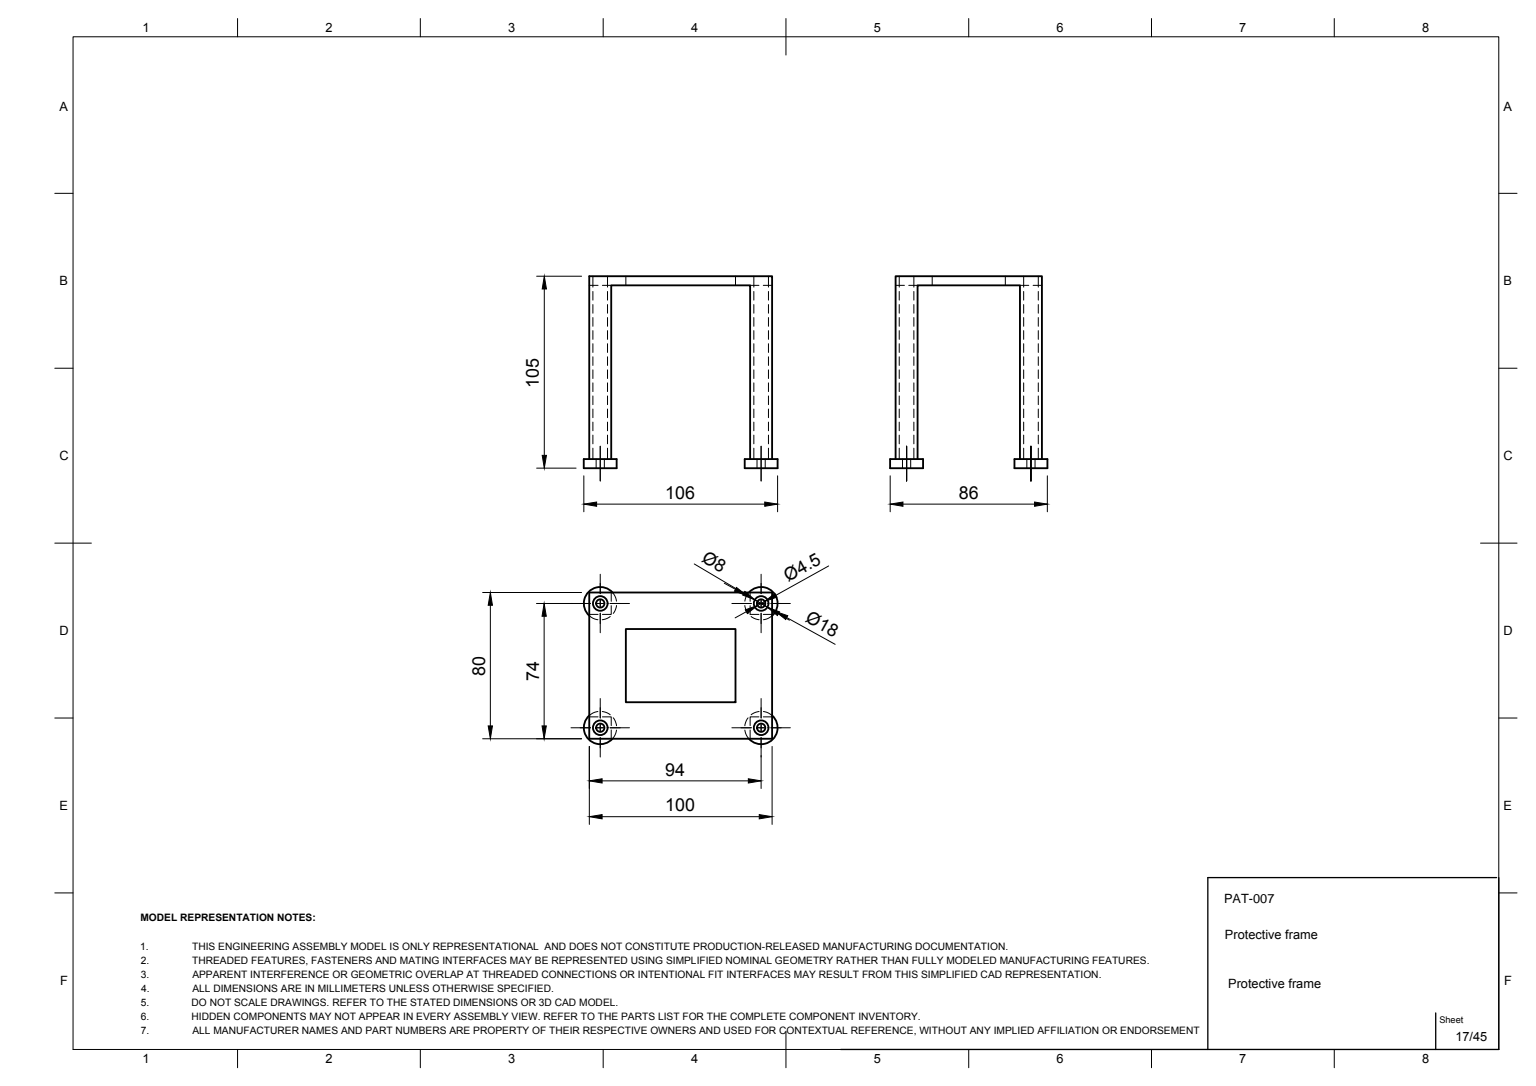
ISO-10303-21;
HEADER;
/* Generated by software containing ST-Developer
 * from STEP Tools, Inc. (www.steptools.com) 
 */

FILE_DESCRIPTION(
/* description */ ('Bearing friction torque test rig'),
/* implementation_level */ '2;1');

FILE_NAME(
/* name */ 'Protective frame.step',
/* time_stamp */ '2026-10-28T03:24:04-07:00',
/* author */ (''),
/* organization */ (''),
/* preprocessor_version */ 'ST-DEVELOPER v20.2',
/* originating_system */ 'Autodesk Translation Framework v15.17.0.0',
/* authorisation */ '');

FILE_SCHEMA (('AUTOMOTIVE_DESIGN { 1 0 10303 214 3 1 1 }'));
ENDSEC;

DATA;
#10=MECHANICAL_DESIGN_GEOMETRIC_PRESENTATION_REPRESENTATION('',(#551),#14822);
#473=SHAPE_REPRESENTATION_RELATIONSHIP('SRR','None',#15012,#512);
#512=ADVANCED_BREP_SHAPE_REPRESENTATION('',(#605),#14792);
#551=STYLED_ITEM('',(#15263),#605);
#605=MANIFOLD_SOLID_BREP('Body1',#7667);
#795=FACE_BOUND('',#1864,.T.);
#796=FACE_BOUND('',#1867,.T.);
#797=FACE_BOUND('',#1873,.T.);
#798=FACE_BOUND('',#1876,.T.);
#799=FACE_BOUND('',#1882,.T.);
#800=FACE_BOUND('',#1885,.T.);
#801=FACE_BOUND('',#1891,.T.);
#802=FACE_BOUND('',#1894,.T.);
#803=FACE_BOUND('',#1904,.T.);
#804=FACE_BOUND('',#1907,.T.);
#805=FACE_BOUND('',#1909,.T.);
#806=FACE_BOUND('',#1911,.T.);
#807=FACE_BOUND('',#1914,.T.);
#808=FACE_BOUND('',#1917,.T.);
#809=FACE_BOUND('',#1918,.T.);
#810=FACE_BOUND('',#1919,.T.);
#811=FACE_BOUND('',#1920,.T.);
#812=FACE_BOUND('',#1921,.T.);
#949=PLANE('',#8521);
#950=PLANE('',#8525);
#951=PLANE('',#8529);
#952=PLANE('',#8530);
#953=PLANE('',#8534);
#954=PLANE('',#8538);
#955=PLANE('',#8542);
#956=PLANE('',#8543);
#957=PLANE('',#8547);
#958=PLANE('',#8551);
#959=PLANE('',#8555);
#960=PLANE('',#8556);
#961=PLANE('',#8560);
#962=PLANE('',#8564);
#963=PLANE('',#8568);
#964=PLANE('',#8569);
#965=PLANE('',#8570);
#966=PLANE('',#8571);
#967=PLANE('',#8572);
#968=PLANE('',#8573);
#969=PLANE('',#8574);
#970=PLANE('',#8575);
#971=PLANE('',#8576);
#972=PLANE('',#8577);
#973=PLANE('',#8578);
#974=PLANE('',#8579);
#975=PLANE('',#8580);
#976=PLANE('',#8581);
#977=PLANE('',#8582);
#978=PLANE('',#8583);
#1266=FACE_OUTER_BOUND('',#1862,.T.);
#1267=FACE_OUTER_BOUND('',#1863,.T.);
#1268=FACE_OUTER_BOUND('',#1865,.T.);
#1269=FACE_OUTER_BOUND('',#1866,.T.);
#1270=FACE_OUTER_BOUND('',#1868,.T.);
#1271=FACE_OUTER_BOUND('',#1869,.T.);
#1272=FACE_OUTER_BOUND('',#1870,.T.);
#1273=FACE_OUTER_BOUND('',#1871,.T.);
#1274=FACE_OUTER_BOUND('',#1872,.T.);
#1275=FACE_OUTER_BOUND('',#1874,.T.);
#1276=FACE_OUTER_BOUND('',#1875,.T.);
#1277=FACE_OUTER_BOUND('',#1877,.T.);
#1278=FACE_OUTER_BOUND('',#1878,.T.);
#1279=FACE_OUTER_BOUND('',#1879,.T.);
#1280=FACE_OUTER_BOUND('',#1880,.T.);
#1281=FACE_OUTER_BOUND('',#1881,.T.);
#1282=FACE_OUTER_BOUND('',#1883,.T.);
#1283=FACE_OUTER_BOUND('',#1884,.T.);
#1284=FACE_OUTER_BOUND('',#1886,.T.);
#1285=FACE_OUTER_BOUND('',#1887,.T.);
#1286=FACE_OUTER_BOUND('',#1888,.T.);
#1287=FACE_OUTER_BOUND('',#1889,.T.);
#1288=FACE_OUTER_BOUND('',#1890,.T.);
#1289=FACE_OUTER_BOUND('',#1892,.T.);
#1290=FACE_OUTER_BOUND('',#1893,.T.);
#1291=FACE_OUTER_BOUND('',#1895,.T.);
#1292=FACE_OUTER_BOUND('',#1896,.T.);
#1293=FACE_OUTER_BOUND('',#1897,.T.);
#1294=FACE_OUTER_BOUND('',#1898,.T.);
#1295=FACE_OUTER_BOUND('',#1899,.T.);
#1296=FACE_OUTER_BOUND('',#1900,.T.);
#1297=FACE_OUTER_BOUND('',#1901,.T.);
#1298=FACE_OUTER_BOUND('',#1902,.T.);
#1299=FACE_OUTER_BOUND('',#1903,.T.);
#1300=FACE_OUTER_BOUND('',#1905,.T.);
#1301=FACE_OUTER_BOUND('',#1906,.T.);
#1302=FACE_OUTER_BOUND('',#1908,.T.);
#1303=FACE_OUTER_BOUND('',#1910,.T.);
#1304=FACE_OUTER_BOUND('',#1912,.T.);
#1305=FACE_OUTER_BOUND('',#1913,.T.);
#1306=FACE_OUTER_BOUND('',#1915,.T.);
#1307=FACE_OUTER_BOUND('',#1916,.T.);
#1862=EDGE_LOOP('',(#5904,#5905,#5906,#5907));
#1863=EDGE_LOOP('',(#5908));
#1864=EDGE_LOOP('',(#5909));
#1865=EDGE_LOOP('',(#5910,#5911,#5912,#5913));
#1866=EDGE_LOOP('',(#5914));
#1867=EDGE_LOOP('',(#5915,#5916,#5917,#5918));
#1868=EDGE_LOOP('',(#5919,#5920,#5921,#5922));
#1869=EDGE_LOOP('',(#5923,#5924,#5925,#5926,#5927,#5928,#5929,#5930));
#1870=EDGE_LOOP('',(#5931,#5932,#5933,#5934,#5935,#5936,#5937,#5938));
#1871=EDGE_LOOP('',(#5939,#5940,#5941,#5942));
#1872=EDGE_LOOP('',(#5943));
#1873=EDGE_LOOP('',(#5944));
#1874=EDGE_LOOP('',(#5945,#5946,#5947,#5948));
#1875=EDGE_LOOP('',(#5949));
#1876=EDGE_LOOP('',(#5950,#5951,#5952,#5953));
#1877=EDGE_LOOP('',(#5954,#5955,#5956,#5957));
#1878=EDGE_LOOP('',(#5958,#5959,#5960,#5961));
#1879=EDGE_LOOP('',(#5962,#5963,#5964,#5965));
#1880=EDGE_LOOP('',(#5966,#5967,#5968,#5969));
#1881=EDGE_LOOP('',(#5970));
#1882=EDGE_LOOP('',(#5971));
#1883=EDGE_LOOP('',(#5972,#5973,#5974,#5975));
#1884=EDGE_LOOP('',(#5976));
#1885=EDGE_LOOP('',(#5977,#5978,#5979,#5980));
#1886=EDGE_LOOP('',(#5981,#5982,#5983,#5984));
#1887=EDGE_LOOP('',(#5985,#5986,#5987,#5988));
#1888=EDGE_LOOP('',(#5989,#5990,#5991,#5992));
#1889=EDGE_LOOP('',(#5993,#5994,#5995,#5996));
#1890=EDGE_LOOP('',(#5997));
#1891=EDGE_LOOP('',(#5998));
#1892=EDGE_LOOP('',(#5999,#6000,#6001,#6002));
#1893=EDGE_LOOP('',(#6003));
#1894=EDGE_LOOP('',(#6004,#6005,#6006,#6007));
#1895=EDGE_LOOP('',(#6008,#6009,#6010,#6011));
#1896=EDGE_LOOP('',(#6012,#6013,#6014,#6015,#6016,#6017,#6018,#6019));
#1897=EDGE_LOOP('',(#6020,#6021,#6022,#6023));
#1898=EDGE_LOOP('',(#6024,#6025,#6026,#6027));
#1899=EDGE_LOOP('',(#6028,#6029,#6030,#6031));
#1900=EDGE_LOOP('',(#6032,#6033,#6034,#6035));
#1901=EDGE_LOOP('',(#6036,#6037,#6038,#6039));
#1902=EDGE_LOOP('',(#6040,#6041,#6042,#6043));
#1903=EDGE_LOOP('',(#6044));
#1904=EDGE_LOOP('',(#6045));
#1905=EDGE_LOOP('',(#6046,#6047,#6048,#6049));
#1906=EDGE_LOOP('',(#6050,#6051,#6052,#6053,#6054,#6055,#6056,#6057,#6058,
#6059,#6060,#6061));
#1907=EDGE_LOOP('',(#6062,#6063,#6064,#6065));
#1908=EDGE_LOOP('',(#6066));
#1909=EDGE_LOOP('',(#6067));
#1910=EDGE_LOOP('',(#6068));
#1911=EDGE_LOOP('',(#6069));
#1912=EDGE_LOOP('',(#6070,#6071,#6072,#6073));
#1913=EDGE_LOOP('',(#6074));
#1914=EDGE_LOOP('',(#6075));
#1915=EDGE_LOOP('',(#6076,#6077,#6078,#6079,#6080,#6081,#6082,#6083));
#1916=EDGE_LOOP('',(#6084,#6085,#6086,#6087));
#1917=EDGE_LOOP('',(#6088));
#1918=EDGE_LOOP('',(#6089));
#1919=EDGE_LOOP('',(#6090));
#1920=EDGE_LOOP('',(#6091));
#1921=EDGE_LOOP('',(#6092,#6093,#6094,#6095));
#2403=LINE('',#12474,#2847);
#2404=LINE('',#12482,#2848);
#2405=LINE('',#12488,#2849);
#2406=LINE('',#12490,#2850);
#2407=LINE('',#12492,#2851);
#2408=LINE('',#12493,#2852);
#2409=LINE('',#12496,#2853);
#2410=LINE('',#12500,#2854);
#2411=LINE('',#12502,#2855);
#2412=LINE('',#12504,#2856);
#2413=LINE('',#12506,#2857);
#2414=LINE('',#12508,#2858);
#2415=LINE('',#12510,#2859);
#2416=LINE('',#12511,#2860);
#2417=LINE('',#12514,#2861);
#2418=LINE('',#12516,#2862);
#2419=LINE('',#12518,#2863);
#2420=LINE('',#12520,#2864);
#2421=LINE('',#12522,#2865);
#2422=LINE('',#12523,#2866);
#2423=LINE('',#12528,#2867);
#2424=LINE('',#12536,#2868);
#2425=LINE('',#12541,#2869);
#2426=LINE('',#12543,#2870);
#2427=LINE('',#12544,#2871);
#2428=LINE('',#12547,#2872);
#2429=LINE('',#12551,#2873);
#2430=LINE('',#12552,#2874);
#2431=LINE('',#12555,#2875);
#2432=LINE('',#12556,#2876);
#2433=LINE('',#12561,#2877);
#2434=LINE('',#12569,#2878);
#2435=LINE('',#12574,#2879);
#2436=LINE('',#12576,#2880);
#2437=LINE('',#12577,#2881);
#2438=LINE('',#12580,#2882);
#2439=LINE('',#12584,#2883);
#2440=LINE('',#12586,#2884);
#2441=LINE('',#12587,#2885);
#2442=LINE('',#12589,#2886);
#2443=LINE('',#12594,#2887);
#2444=LINE('',#12602,#2888);
#2445=LINE('',#12608,#2889);
#2446=LINE('',#12610,#2890);
#2447=LINE('',#12612,#2891);
#2448=LINE('',#12613,#2892);
#2449=LINE('',#12616,#2893);
#2450=LINE('',#12620,#2894);
#2451=LINE('',#12621,#2895);
#2452=LINE('',#12623,#2896);
#2453=LINE('',#12624,#2897);
#2454=LINE('',#12627,#2898);
#2455=LINE('',#12628,#2899);
#2456=LINE('',#12632,#2900);
#2457=LINE('',#12634,#2901);
#2458=LINE('',#12636,#2902);
#2459=LINE('',#12637,#2903);
#2460=LINE('',#12640,#2904);
#2461=LINE('',#12642,#2905);
#2462=LINE('',#12643,#2906);
#2463=LINE('',#12646,#2907);
#2464=LINE('',#12648,#2908);
#2465=LINE('',#12649,#2909);
#2466=LINE('',#12651,#2910);
#2467=LINE('',#12652,#2911);
#2468=LINE('',#12655,#2912);
#2469=LINE('',#12656,#2913);
#2470=LINE('',#12659,#2914);
#2471=LINE('',#12662,#2915);
#2472=LINE('',#12663,#2916);
#2473=LINE('',#12667,#2917);
#2474=LINE('',#12670,#2918);
#2847=VECTOR('',#10106,0.4);
#2848=VECTOR('',#10117,0.225);
#2849=VECTOR('',#10122,1.);
#2850=VECTOR('',#10123,1.);
#2851=VECTOR('',#10124,1.);
#2852=VECTOR('',#10125,1.);
#2853=VECTOR('',#10128,0.9);
#2854=VECTOR('',#10133,1.);
#2855=VECTOR('',#10134,1.);
#2856=VECTOR('',#10135,1.);
#2857=VECTOR('',#10136,1.);
#2858=VECTOR('',#10137,1.);
#2859=VECTOR('',#10138,1.);
#2860=VECTOR('',#10139,1.);
#2861=VECTOR('',#10142,1.);
#2862=VECTOR('',#10143,1.);
#2863=VECTOR('',#10144,1.);
#2864=VECTOR('',#10145,1.);
#2865=VECTOR('',#10146,1.);
#2866=VECTOR('',#10147,1.);
#2867=VECTOR('',#10152,0.4);
#2868=VECTOR('',#10163,0.225);
#2869=VECTOR('',#10168,1.);
#2870=VECTOR('',#10169,1.);
#2871=VECTOR('',#10170,1.);
#2872=VECTOR('',#10173,0.9);
#2873=VECTOR('',#10178,1.);
#2874=VECTOR('',#10179,1.);
#2875=VECTOR('',#10182,1.);
#2876=VECTOR('',#10183,1.);
#2877=VECTOR('',#10188,0.4);
#2878=VECTOR('',#10199,0.225);
#2879=VECTOR('',#10204,1.);
#2880=VECTOR('',#10205,1.);
#2881=VECTOR('',#10206,1.);
#2882=VECTOR('',#10209,0.9);
#2883=VECTOR('',#10214,1.);
#2884=VECTOR('',#10215,1.);
#2885=VECTOR('',#10216,1.);
#2886=VECTOR('',#10219,1.);
#2887=VECTOR('',#10224,0.4);
#2888=VECTOR('',#10235,0.225);
#2889=VECTOR('',#10240,1.);
#2890=VECTOR('',#10241,1.);
#2891=VECTOR('',#10242,1.);
#2892=VECTOR('',#10243,1.);
#2893=VECTOR('',#10246,0.9);
#2894=VECTOR('',#10251,1.);
#2895=VECTOR('',#10252,1.);
#2896=VECTOR('',#10253,1.);
#2897=VECTOR('',#10254,1.);
#2898=VECTOR('',#10257,1.);
#2899=VECTOR('',#10258,1.);
#2900=VECTOR('',#10261,1.);
#2901=VECTOR('',#10262,1.);
#2902=VECTOR('',#10263,1.);
#2903=VECTOR('',#10264,1.);
#2904=VECTOR('',#10267,1.);
#2905=VECTOR('',#10268,1.);
#2906=VECTOR('',#10269,1.);
#2907=VECTOR('',#10272,1.);
#2908=VECTOR('',#10273,1.);
#2909=VECTOR('',#10274,1.);
#2910=VECTOR('',#10277,1.);
#2911=VECTOR('',#10278,1.);
#2912=VECTOR('',#10281,1.);
#2913=VECTOR('',#10282,1.);
#2914=VECTOR('',#10287,1.);
#2915=VECTOR('',#10290,1.);
#2916=VECTOR('',#10291,1.);
#2917=VECTOR('',#10298,1.);
#2918=VECTOR('',#10303,1.);
#3295=CIRCLE('',#8519,0.4);
#3296=CIRCLE('',#8520,0.4);
#3297=CIRCLE('',#8522,0.225);
#3298=CIRCLE('',#8524,0.225);
#3299=CIRCLE('',#8526,0.9);
#3300=CIRCLE('',#8528,0.9);
#3301=CIRCLE('',#8532,0.4);
#3302=CIRCLE('',#8533,0.4);
#3303=CIRCLE('',#8535,0.225);
#3304=CIRCLE('',#8537,0.225);
#3305=CIRCLE('',#8539,0.9);
#3306=CIRCLE('',#8541,0.9);
#3307=CIRCLE('',#8545,0.4);
#3308=CIRCLE('',#8546,0.4);
#3309=CIRCLE('',#8548,0.225);
#3310=CIRCLE('',#8550,0.225);
#3311=CIRCLE('',#8552,0.9);
#3312=CIRCLE('',#8554,0.9);
#3313=CIRCLE('',#8558,0.4);
#3314=CIRCLE('',#8559,0.4);
#3315=CIRCLE('',#8561,0.225);
#3316=CIRCLE('',#8563,0.225);
#3317=CIRCLE('',#8565,0.9);
#3318=CIRCLE('',#8567,0.9);
#3805=VERTEX_POINT('',#12471);
#3806=VERTEX_POINT('',#12473);
#3807=VERTEX_POINT('',#12477);
#3808=VERTEX_POINT('',#12480);
#3809=VERTEX_POINT('',#12484);
#3810=VERTEX_POINT('',#12486);
#3811=VERTEX_POINT('',#12487);
#3812=VERTEX_POINT('',#12489);
#3813=VERTEX_POINT('',#12491);
#3814=VERTEX_POINT('',#12495);
#3815=VERTEX_POINT('',#12499);
#3816=VERTEX_POINT('',#12501);
#3817=VERTEX_POINT('',#12503);
#3818=VERTEX_POINT('',#12505);
#3819=VERTEX_POINT('',#12507);
#3820=VERTEX_POINT('',#12509);
#3821=VERTEX_POINT('',#12513);
#3822=VERTEX_POINT('',#12515);
#3823=VERTEX_POINT('',#12517);
#3824=VERTEX_POINT('',#12519);
#3825=VERTEX_POINT('',#12521);
#3826=VERTEX_POINT('',#12525);
#3827=VERTEX_POINT('',#12527);
#3828=VERTEX_POINT('',#12531);
#3829=VERTEX_POINT('',#12534);
#3830=VERTEX_POINT('',#12538);
#3831=VERTEX_POINT('',#12540);
#3832=VERTEX_POINT('',#12542);
#3833=VERTEX_POINT('',#12546);
#3834=VERTEX_POINT('',#12550);
#3835=VERTEX_POINT('',#12554);
#3836=VERTEX_POINT('',#12558);
#3837=VERTEX_POINT('',#12560);
#3838=VERTEX_POINT('',#12564);
#3839=VERTEX_POINT('',#12567);
#3840=VERTEX_POINT('',#12571);
#3841=VERTEX_POINT('',#12573);
#3842=VERTEX_POINT('',#12575);
#3843=VERTEX_POINT('',#12579);
#3844=VERTEX_POINT('',#12583);
#3845=VERTEX_POINT('',#12585);
#3846=VERTEX_POINT('',#12591);
#3847=VERTEX_POINT('',#12593);
#3848=VERTEX_POINT('',#12597);
#3849=VERTEX_POINT('',#12600);
#3850=VERTEX_POINT('',#12604);
#3851=VERTEX_POINT('',#12606);
#3852=VERTEX_POINT('',#12607);
#3853=VERTEX_POINT('',#12609);
#3854=VERTEX_POINT('',#12611);
#3855=VERTEX_POINT('',#12615);
#3856=VERTEX_POINT('',#12619);
#3857=VERTEX_POINT('',#12622);
#3858=VERTEX_POINT('',#12626);
#3859=VERTEX_POINT('',#12630);
#3860=VERTEX_POINT('',#12631);
#3861=VERTEX_POINT('',#12633);
#3862=VERTEX_POINT('',#12635);
#3863=VERTEX_POINT('',#12639);
#3864=VERTEX_POINT('',#12641);
#3865=VERTEX_POINT('',#12645);
#3866=VERTEX_POINT('',#12647);
#3867=VERTEX_POINT('',#12654);
#3868=VERTEX_POINT('',#12661);
#4578=EDGE_CURVE('',#3805,#3805,#3295,.T.);
#4579=EDGE_CURVE('',#3805,#3806,#2403,.T.);
#4580=EDGE_CURVE('',#3806,#3806,#3296,.T.);
#4581=EDGE_CURVE('',#3807,#3807,#3297,.T.);
#4582=EDGE_CURVE('',#3808,#3808,#3298,.T.);
#4583=EDGE_CURVE('',#3808,#3807,#2404,.T.);
#4584=EDGE_CURVE('',#3809,#3809,#3299,.T.);
#4585=EDGE_CURVE('',#3810,#3811,#2405,.T.);
#4586=EDGE_CURVE('',#3812,#3810,#2406,.T.);
#4587=EDGE_CURVE('',#3813,#3812,#2407,.T.);
#4588=EDGE_CURVE('',#3811,#3813,#2408,.T.);
#4589=EDGE_CURVE('',#3809,#3814,#2409,.T.);
#4590=EDGE_CURVE('',#3814,#3814,#3300,.T.);
#4591=EDGE_CURVE('',#3812,#3815,#2410,.T.);
#4592=EDGE_CURVE('',#3816,#3815,#2411,.T.);
#4593=EDGE_CURVE('',#3817,#3816,#2412,.T.);
#4594=EDGE_CURVE('',#3817,#3818,#2413,.T.);
#4595=EDGE_CURVE('',#3819,#3818,#2414,.T.);
#4596=EDGE_CURVE('',#3819,#3820,#2415,.T.);
#4597=EDGE_CURVE('',#3813,#3820,#2416,.T.);
#4598=EDGE_CURVE('',#3810,#3821,#2417,.T.);
#4599=EDGE_CURVE('',#3821,#3822,#2418,.T.);
#4600=EDGE_CURVE('',#3822,#3823,#2419,.T.);
#4601=EDGE_CURVE('',#3823,#3824,#2420,.T.);
#4602=EDGE_CURVE('',#3824,#3825,#2421,.T.);
#4603=EDGE_CURVE('',#3815,#3825,#2422,.T.);
#4604=EDGE_CURVE('',#3826,#3826,#3301,.T.);
#4605=EDGE_CURVE('',#3826,#3827,#2423,.T.);
#4606=EDGE_CURVE('',#3827,#3827,#3302,.T.);
#4607=EDGE_CURVE('',#3828,#3828,#3303,.T.);
#4608=EDGE_CURVE('',#3829,#3829,#3304,.T.);
#4609=EDGE_CURVE('',#3829,#3828,#2424,.T.);
#4610=EDGE_CURVE('',#3830,#3830,#3305,.T.);
#4611=EDGE_CURVE('',#3831,#3817,#2425,.T.);
#4612=EDGE_CURVE('',#3832,#3831,#2426,.T.);
#4613=EDGE_CURVE('',#3818,#3832,#2427,.T.);
#4614=EDGE_CURVE('',#3830,#3833,#2428,.T.);
#4615=EDGE_CURVE('',#3833,#3833,#3306,.T.);
#4616=EDGE_CURVE('',#3832,#3834,#2429,.T.);
#4617=EDGE_CURVE('',#3819,#3834,#2430,.T.);
#4618=EDGE_CURVE('',#3835,#3831,#2431,.T.);
#4619=EDGE_CURVE('',#3834,#3835,#2432,.T.);
#4620=EDGE_CURVE('',#3836,#3836,#3307,.T.);
#4621=EDGE_CURVE('',#3836,#3837,#2433,.T.);
#4622=EDGE_CURVE('',#3837,#3837,#3308,.T.);
#4623=EDGE_CURVE('',#3838,#3838,#3309,.T.);
#4624=EDGE_CURVE('',#3839,#3839,#3310,.T.);
#4625=EDGE_CURVE('',#3839,#3838,#2434,.T.);
#4626=EDGE_CURVE('',#3840,#3840,#3311,.T.);
#4627=EDGE_CURVE('',#3841,#3823,#2435,.T.);
#4628=EDGE_CURVE('',#3842,#3841,#2436,.T.);
#4629=EDGE_CURVE('',#3824,#3842,#2437,.T.);
#4630=EDGE_CURVE('',#3840,#3843,#2438,.T.);
#4631=EDGE_CURVE('',#3843,#3843,#3312,.T.);
#4632=EDGE_CURVE('',#3841,#3844,#2439,.T.);
#4633=EDGE_CURVE('',#3845,#3844,#2440,.T.);
#4634=EDGE_CURVE('',#3845,#3842,#2441,.T.);
#4635=EDGE_CURVE('',#3844,#3822,#2442,.T.);
#4636=EDGE_CURVE('',#3846,#3846,#3313,.T.);
#4637=EDGE_CURVE('',#3846,#3847,#2443,.T.);
#4638=EDGE_CURVE('',#3847,#3847,#3314,.T.);
#4639=EDGE_CURVE('',#3848,#3848,#3315,.T.);
#4640=EDGE_CURVE('',#3849,#3849,#3316,.T.);
#4641=EDGE_CURVE('',#3849,#3848,#2444,.T.);
#4642=EDGE_CURVE('',#3850,#3850,#3317,.T.);
#4643=EDGE_CURVE('',#3851,#3852,#2445,.T.);
#4644=EDGE_CURVE('',#3853,#3851,#2446,.T.);
#4645=EDGE_CURVE('',#3854,#3853,#2447,.T.);
#4646=EDGE_CURVE('',#3852,#3854,#2448,.T.);
#4647=EDGE_CURVE('',#3850,#3855,#2449,.T.);
#4648=EDGE_CURVE('',#3855,#3855,#3318,.T.);
#4649=EDGE_CURVE('',#3856,#3816,#2450,.T.);
#4650=EDGE_CURVE('',#3854,#3856,#2451,.T.);
#4651=EDGE_CURVE('',#3853,#3857,#2452,.T.);
#4652=EDGE_CURVE('',#3857,#3835,#2453,.T.);
#4653=EDGE_CURVE('',#3858,#3851,#2454,.T.);
#4654=EDGE_CURVE('',#3857,#3858,#2455,.T.);
#4655=EDGE_CURVE('',#3859,#3860,#2456,.T.);
#4656=EDGE_CURVE('',#3859,#3861,#2457,.T.);
#4657=EDGE_CURVE('',#3862,#3861,#2458,.T.);
#4658=EDGE_CURVE('',#3860,#3862,#2459,.T.);
#4659=EDGE_CURVE('',#3860,#3863,#2460,.T.);
#4660=EDGE_CURVE('',#3864,#3862,#2461,.T.);
#4661=EDGE_CURVE('',#3863,#3864,#2462,.T.);
#4662=EDGE_CURVE('',#3863,#3865,#2463,.T.);
#4663=EDGE_CURVE('',#3866,#3864,#2464,.T.);
#4664=EDGE_CURVE('',#3865,#3866,#2465,.T.);
#4665=EDGE_CURVE('',#3865,#3859,#2466,.T.);
#4666=EDGE_CURVE('',#3861,#3866,#2467,.T.);
#4667=EDGE_CURVE('',#3867,#3811,#2468,.T.);
#4668=EDGE_CURVE('',#3821,#3867,#2469,.T.);
#4669=EDGE_CURVE('',#3867,#3820,#2470,.T.);
#4670=EDGE_CURVE('',#3858,#3868,#2471,.T.);
#4671=EDGE_CURVE('',#3845,#3868,#2472,.T.);
#4672=EDGE_CURVE('',#3852,#3868,#2473,.T.);
#4673=EDGE_CURVE('',#3825,#3856,#2474,.T.);
#5904=ORIENTED_EDGE('',*,*,#4578,.F.);
#5905=ORIENTED_EDGE('',*,*,#4579,.T.);
#5906=ORIENTED_EDGE('',*,*,#4580,.F.);
#5907=ORIENTED_EDGE('',*,*,#4579,.F.);
#5908=ORIENTED_EDGE('',*,*,#4578,.T.);
#5909=ORIENTED_EDGE('',*,*,#4581,.F.);
#5910=ORIENTED_EDGE('',*,*,#4582,.F.);
#5911=ORIENTED_EDGE('',*,*,#4583,.T.);
#5912=ORIENTED_EDGE('',*,*,#4581,.T.);
#5913=ORIENTED_EDGE('',*,*,#4583,.F.);
#5914=ORIENTED_EDGE('',*,*,#4584,.T.);
#5915=ORIENTED_EDGE('',*,*,#4585,.F.);
#5916=ORIENTED_EDGE('',*,*,#4586,.F.);
#5917=ORIENTED_EDGE('',*,*,#4587,.F.);
#5918=ORIENTED_EDGE('',*,*,#4588,.F.);
#5919=ORIENTED_EDGE('',*,*,#4584,.F.);
#5920=ORIENTED_EDGE('',*,*,#4589,.T.);
#5921=ORIENTED_EDGE('',*,*,#4590,.T.);
#5922=ORIENTED_EDGE('',*,*,#4589,.F.);
#5923=ORIENTED_EDGE('',*,*,#4587,.T.);
#5924=ORIENTED_EDGE('',*,*,#4591,.T.);
#5925=ORIENTED_EDGE('',*,*,#4592,.F.);
#5926=ORIENTED_EDGE('',*,*,#4593,.F.);
#5927=ORIENTED_EDGE('',*,*,#4594,.T.);
#5928=ORIENTED_EDGE('',*,*,#4595,.F.);
#5929=ORIENTED_EDGE('',*,*,#4596,.T.);
#5930=ORIENTED_EDGE('',*,*,#4597,.F.);
#5931=ORIENTED_EDGE('',*,*,#4586,.T.);
#5932=ORIENTED_EDGE('',*,*,#4598,.T.);
#5933=ORIENTED_EDGE('',*,*,#4599,.T.);
#5934=ORIENTED_EDGE('',*,*,#4600,.T.);
#5935=ORIENTED_EDGE('',*,*,#4601,.T.);
#5936=ORIENTED_EDGE('',*,*,#4602,.T.);
#5937=ORIENTED_EDGE('',*,*,#4603,.F.);
#5938=ORIENTED_EDGE('',*,*,#4591,.F.);
#5939=ORIENTED_EDGE('',*,*,#4604,.F.);
#5940=ORIENTED_EDGE('',*,*,#4605,.T.);
#5941=ORIENTED_EDGE('',*,*,#4606,.F.);
#5942=ORIENTED_EDGE('',*,*,#4605,.F.);
#5943=ORIENTED_EDGE('',*,*,#4604,.T.);
#5944=ORIENTED_EDGE('',*,*,#4607,.F.);
#5945=ORIENTED_EDGE('',*,*,#4608,.F.);
#5946=ORIENTED_EDGE('',*,*,#4609,.T.);
#5947=ORIENTED_EDGE('',*,*,#4607,.T.);
#5948=ORIENTED_EDGE('',*,*,#4609,.F.);
#5949=ORIENTED_EDGE('',*,*,#4610,.T.);
#5950=ORIENTED_EDGE('',*,*,#4611,.F.);
#5951=ORIENTED_EDGE('',*,*,#4612,.F.);
#5952=ORIENTED_EDGE('',*,*,#4613,.F.);
#5953=ORIENTED_EDGE('',*,*,#4594,.F.);
#5954=ORIENTED_EDGE('',*,*,#4610,.F.);
#5955=ORIENTED_EDGE('',*,*,#4614,.T.);
#5956=ORIENTED_EDGE('',*,*,#4615,.T.);
#5957=ORIENTED_EDGE('',*,*,#4614,.F.);
#5958=ORIENTED_EDGE('',*,*,#4613,.T.);
#5959=ORIENTED_EDGE('',*,*,#4616,.T.);
#5960=ORIENTED_EDGE('',*,*,#4617,.F.);
#5961=ORIENTED_EDGE('',*,*,#4595,.T.);
#5962=ORIENTED_EDGE('',*,*,#4612,.T.);
#5963=ORIENTED_EDGE('',*,*,#4618,.F.);
#5964=ORIENTED_EDGE('',*,*,#4619,.F.);
#5965=ORIENTED_EDGE('',*,*,#4616,.F.);
#5966=ORIENTED_EDGE('',*,*,#4620,.F.);
#5967=ORIENTED_EDGE('',*,*,#4621,.T.);
#5968=ORIENTED_EDGE('',*,*,#4622,.F.);
#5969=ORIENTED_EDGE('',*,*,#4621,.F.);
#5970=ORIENTED_EDGE('',*,*,#4620,.T.);
#5971=ORIENTED_EDGE('',*,*,#4623,.F.);
#5972=ORIENTED_EDGE('',*,*,#4624,.F.);
#5973=ORIENTED_EDGE('',*,*,#4625,.T.);
#5974=ORIENTED_EDGE('',*,*,#4623,.T.);
#5975=ORIENTED_EDGE('',*,*,#4625,.F.);
#5976=ORIENTED_EDGE('',*,*,#4626,.T.);
#5977=ORIENTED_EDGE('',*,*,#4601,.F.);
#5978=ORIENTED_EDGE('',*,*,#4627,.F.);
#5979=ORIENTED_EDGE('',*,*,#4628,.F.);
#5980=ORIENTED_EDGE('',*,*,#4629,.F.);
#5981=ORIENTED_EDGE('',*,*,#4626,.F.);
#5982=ORIENTED_EDGE('',*,*,#4630,.T.);
#5983=ORIENTED_EDGE('',*,*,#4631,.T.);
#5984=ORIENTED_EDGE('',*,*,#4630,.F.);
#5985=ORIENTED_EDGE('',*,*,#4628,.T.);
#5986=ORIENTED_EDGE('',*,*,#4632,.T.);
#5987=ORIENTED_EDGE('',*,*,#4633,.F.);
#5988=ORIENTED_EDGE('',*,*,#4634,.T.);
#5989=ORIENTED_EDGE('',*,*,#4627,.T.);
#5990=ORIENTED_EDGE('',*,*,#4600,.F.);
#5991=ORIENTED_EDGE('',*,*,#4635,.F.);
#5992=ORIENTED_EDGE('',*,*,#4632,.F.);
#5993=ORIENTED_EDGE('',*,*,#4636,.F.);
#5994=ORIENTED_EDGE('',*,*,#4637,.T.);
#5995=ORIENTED_EDGE('',*,*,#4638,.F.);
#5996=ORIENTED_EDGE('',*,*,#4637,.F.);
#5997=ORIENTED_EDGE('',*,*,#4636,.T.);
#5998=ORIENTED_EDGE('',*,*,#4639,.F.);
#5999=ORIENTED_EDGE('',*,*,#4640,.F.);
#6000=ORIENTED_EDGE('',*,*,#4641,.T.);
#6001=ORIENTED_EDGE('',*,*,#4639,.T.);
#6002=ORIENTED_EDGE('',*,*,#4641,.F.);
#6003=ORIENTED_EDGE('',*,*,#4642,.T.);
#6004=ORIENTED_EDGE('',*,*,#4643,.F.);
#6005=ORIENTED_EDGE('',*,*,#4644,.F.);
#6006=ORIENTED_EDGE('',*,*,#4645,.F.);
#6007=ORIENTED_EDGE('',*,*,#4646,.F.);
#6008=ORIENTED_EDGE('',*,*,#4642,.F.);
#6009=ORIENTED_EDGE('',*,*,#4647,.T.);
#6010=ORIENTED_EDGE('',*,*,#4648,.T.);
#6011=ORIENTED_EDGE('',*,*,#4647,.F.);
#6012=ORIENTED_EDGE('',*,*,#4611,.T.);
#6013=ORIENTED_EDGE('',*,*,#4593,.T.);
#6014=ORIENTED_EDGE('',*,*,#4649,.F.);
#6015=ORIENTED_EDGE('',*,*,#4650,.F.);
#6016=ORIENTED_EDGE('',*,*,#4645,.T.);
#6017=ORIENTED_EDGE('',*,*,#4651,.T.);
#6018=ORIENTED_EDGE('',*,*,#4652,.T.);
#6019=ORIENTED_EDGE('',*,*,#4618,.T.);
#6020=ORIENTED_EDGE('',*,*,#4644,.T.);
#6021=ORIENTED_EDGE('',*,*,#4653,.F.);
#6022=ORIENTED_EDGE('',*,*,#4654,.F.);
#6023=ORIENTED_EDGE('',*,*,#4651,.F.);
#6024=ORIENTED_EDGE('',*,*,#4655,.F.);
#6025=ORIENTED_EDGE('',*,*,#4656,.T.);
#6026=ORIENTED_EDGE('',*,*,#4657,.F.);
#6027=ORIENTED_EDGE('',*,*,#4658,.F.);
#6028=ORIENTED_EDGE('',*,*,#4659,.F.);
#6029=ORIENTED_EDGE('',*,*,#4658,.T.);
#6030=ORIENTED_EDGE('',*,*,#4660,.F.);
#6031=ORIENTED_EDGE('',*,*,#4661,.F.);
#6032=ORIENTED_EDGE('',*,*,#4662,.F.);
#6033=ORIENTED_EDGE('',*,*,#4661,.T.);
#6034=ORIENTED_EDGE('',*,*,#4663,.F.);
#6035=ORIENTED_EDGE('',*,*,#4664,.F.);
#6036=ORIENTED_EDGE('',*,*,#4665,.F.);
#6037=ORIENTED_EDGE('',*,*,#4664,.T.);
#6038=ORIENTED_EDGE('',*,*,#4666,.F.);
#6039=ORIENTED_EDGE('',*,*,#4656,.F.);
#6040=ORIENTED_EDGE('',*,*,#4585,.T.);
#6041=ORIENTED_EDGE('',*,*,#4667,.F.);
#6042=ORIENTED_EDGE('',*,*,#4668,.F.);
#6043=ORIENTED_EDGE('',*,*,#4598,.F.);
#6044=ORIENTED_EDGE('',*,*,#4590,.F.);
#6045=ORIENTED_EDGE('',*,*,#4582,.T.);
#6046=ORIENTED_EDGE('',*,*,#4588,.T.);
#6047=ORIENTED_EDGE('',*,*,#4597,.T.);
#6048=ORIENTED_EDGE('',*,*,#4669,.F.);
#6049=ORIENTED_EDGE('',*,*,#4667,.T.);
#6050=ORIENTED_EDGE('',*,*,#4668,.T.);
#6051=ORIENTED_EDGE('',*,*,#4669,.T.);
#6052=ORIENTED_EDGE('',*,*,#4596,.F.);
#6053=ORIENTED_EDGE('',*,*,#4617,.T.);
#6054=ORIENTED_EDGE('',*,*,#4619,.T.);
#6055=ORIENTED_EDGE('',*,*,#4652,.F.);
#6056=ORIENTED_EDGE('',*,*,#4654,.T.);
#6057=ORIENTED_EDGE('',*,*,#4670,.T.);
#6058=ORIENTED_EDGE('',*,*,#4671,.F.);
#6059=ORIENTED_EDGE('',*,*,#4633,.T.);
#6060=ORIENTED_EDGE('',*,*,#4635,.T.);
#6061=ORIENTED_EDGE('',*,*,#4599,.F.);
#6062=ORIENTED_EDGE('',*,*,#4662,.T.);
#6063=ORIENTED_EDGE('',*,*,#4665,.T.);
#6064=ORIENTED_EDGE('',*,*,#4655,.T.);
#6065=ORIENTED_EDGE('',*,*,#4659,.T.);
#6066=ORIENTED_EDGE('',*,*,#4615,.F.);
#6067=ORIENTED_EDGE('',*,*,#4608,.T.);
#6068=ORIENTED_EDGE('',*,*,#4631,.F.);
#6069=ORIENTED_EDGE('',*,*,#4624,.T.);
#6070=ORIENTED_EDGE('',*,*,#4643,.T.);
#6071=ORIENTED_EDGE('',*,*,#4672,.T.);
#6072=ORIENTED_EDGE('',*,*,#4670,.F.);
#6073=ORIENTED_EDGE('',*,*,#4653,.T.);
#6074=ORIENTED_EDGE('',*,*,#4648,.F.);
#6075=ORIENTED_EDGE('',*,*,#4640,.T.);
#6076=ORIENTED_EDGE('',*,*,#4629,.T.);
#6077=ORIENTED_EDGE('',*,*,#4634,.F.);
#6078=ORIENTED_EDGE('',*,*,#4671,.T.);
#6079=ORIENTED_EDGE('',*,*,#4672,.F.);
#6080=ORIENTED_EDGE('',*,*,#4646,.T.);
#6081=ORIENTED_EDGE('',*,*,#4650,.T.);
#6082=ORIENTED_EDGE('',*,*,#4673,.F.);
#6083=ORIENTED_EDGE('',*,*,#4602,.F.);
#6084=ORIENTED_EDGE('',*,*,#4673,.T.);
#6085=ORIENTED_EDGE('',*,*,#4649,.T.);
#6086=ORIENTED_EDGE('',*,*,#4592,.T.);
#6087=ORIENTED_EDGE('',*,*,#4603,.T.);
#6088=ORIENTED_EDGE('',*,*,#4580,.T.);
#6089=ORIENTED_EDGE('',*,*,#4606,.T.);
#6090=ORIENTED_EDGE('',*,*,#4622,.T.);
#6091=ORIENTED_EDGE('',*,*,#4638,.T.);
#6092=ORIENTED_EDGE('',*,*,#4663,.T.);
#6093=ORIENTED_EDGE('',*,*,#4660,.T.);
#6094=ORIENTED_EDGE('',*,*,#4657,.T.);
#6095=ORIENTED_EDGE('',*,*,#4666,.T.);
#7136=CYLINDRICAL_SURFACE('',#8518,0.4);
#7137=CYLINDRICAL_SURFACE('',#8523,0.225);
#7138=CYLINDRICAL_SURFACE('',#8527,0.9);
#7139=CYLINDRICAL_SURFACE('',#8531,0.4);
#7140=CYLINDRICAL_SURFACE('',#8536,0.225);
#7141=CYLINDRICAL_SURFACE('',#8540,0.9);
#7142=CYLINDRICAL_SURFACE('',#8544,0.4);
#7143=CYLINDRICAL_SURFACE('',#8549,0.225);
#7144=CYLINDRICAL_SURFACE('',#8553,0.9);
#7145=CYLINDRICAL_SURFACE('',#8557,0.4);
#7146=CYLINDRICAL_SURFACE('',#8562,0.225);
#7147=CYLINDRICAL_SURFACE('',#8566,0.9);
#7377=ADVANCED_FACE('',(#1266),#7136,.F.);
#7378=ADVANCED_FACE('',(#1267,#795),#949,.T.);
#7379=ADVANCED_FACE('',(#1268),#7137,.F.);
#7380=ADVANCED_FACE('',(#1269,#796),#950,.T.);
#7381=ADVANCED_FACE('',(#1270),#7138,.T.);
#7382=ADVANCED_FACE('',(#1271),#951,.T.);
#7383=ADVANCED_FACE('',(#1272),#952,.T.);
#7384=ADVANCED_FACE('',(#1273),#7139,.F.);
#7385=ADVANCED_FACE('',(#1274,#797),#953,.T.);
#7386=ADVANCED_FACE('',(#1275),#7140,.F.);
#7387=ADVANCED_FACE('',(#1276,#798),#954,.T.);
#7388=ADVANCED_FACE('',(#1277),#7141,.T.);
#7389=ADVANCED_FACE('',(#1278),#955,.T.);
#7390=ADVANCED_FACE('',(#1279),#956,.T.);
#7391=ADVANCED_FACE('',(#1280),#7142,.F.);
#7392=ADVANCED_FACE('',(#1281,#799),#957,.T.);
#7393=ADVANCED_FACE('',(#1282),#7143,.F.);
#7394=ADVANCED_FACE('',(#1283,#800),#958,.T.);
#7395=ADVANCED_FACE('',(#1284),#7144,.T.);
#7396=ADVANCED_FACE('',(#1285),#959,.F.);
#7397=ADVANCED_FACE('',(#1286),#960,.T.);
#7398=ADVANCED_FACE('',(#1287),#7145,.F.);
#7399=ADVANCED_FACE('',(#1288,#801),#961,.T.);
#7400=ADVANCED_FACE('',(#1289),#7146,.F.);
#7401=ADVANCED_FACE('',(#1290,#802),#962,.T.);
#7402=ADVANCED_FACE('',(#1291),#7147,.T.);
#7403=ADVANCED_FACE('',(#1292),#963,.T.);
#7404=ADVANCED_FACE('',(#1293),#964,.T.);
#7405=ADVANCED_FACE('',(#1294),#965,.F.);
#7406=ADVANCED_FACE('',(#1295),#966,.F.);
#7407=ADVANCED_FACE('',(#1296),#967,.F.);
#7408=ADVANCED_FACE('',(#1297),#968,.F.);
#7409=ADVANCED_FACE('',(#1298),#969,.T.);
#7410=ADVANCED_FACE('',(#1299,#803),#970,.T.);
#7411=ADVANCED_FACE('',(#1300),#971,.F.);
#7412=ADVANCED_FACE('',(#1301,#804),#972,.F.);
#7413=ADVANCED_FACE('',(#1302,#805),#973,.T.);
#7414=ADVANCED_FACE('',(#1303,#806),#974,.T.);
#7415=ADVANCED_FACE('',(#1304),#975,.T.);
#7416=ADVANCED_FACE('',(#1305,#807),#976,.T.);
#7417=ADVANCED_FACE('',(#1306),#977,.T.);
#7418=ADVANCED_FACE('',(#1307,#808,#809,#810,#811,#812),#978,.T.);
#7667=CLOSED_SHELL('',(#7377,#7378,#7379,#7380,#7381,#7382,#7383,#7384,
#7385,#7386,#7387,#7388,#7389,#7390,#7391,#7392,#7393,#7394,#7395,#7396,
#7397,#7398,#7399,#7400,#7401,#7402,#7403,#7404,#7405,#7406,#7407,#7408,
#7409,#7410,#7411,#7412,#7413,#7414,#7415,#7416,#7417,#7418));
#8517=AXIS2_PLACEMENT_3D('',#12469,#10100,#10101);
#8518=AXIS2_PLACEMENT_3D('',#12470,#10102,#10103);
#8519=AXIS2_PLACEMENT_3D('',#12472,#10104,#10105);
#8520=AXIS2_PLACEMENT_3D('',#12475,#10107,#10108);
#8521=AXIS2_PLACEMENT_3D('',#12476,#10109,#10110);
#8522=AXIS2_PLACEMENT_3D('',#12478,#10111,#10112);
#8523=AXIS2_PLACEMENT_3D('',#12479,#10113,#10114);
#8524=AXIS2_PLACEMENT_3D('',#12481,#10115,#10116);
#8525=AXIS2_PLACEMENT_3D('',#12483,#10118,#10119);
#8526=AXIS2_PLACEMENT_3D('',#12485,#10120,#10121);
#8527=AXIS2_PLACEMENT_3D('',#12494,#10126,#10127);
#8528=AXIS2_PLACEMENT_3D('',#12497,#10129,#10130);
#8529=AXIS2_PLACEMENT_3D('',#12498,#10131,#10132);
#8530=AXIS2_PLACEMENT_3D('',#12512,#10140,#10141);
#8531=AXIS2_PLACEMENT_3D('',#12524,#10148,#10149);
#8532=AXIS2_PLACEMENT_3D('',#12526,#10150,#10151);
#8533=AXIS2_PLACEMENT_3D('',#12529,#10153,#10154);
#8534=AXIS2_PLACEMENT_3D('',#12530,#10155,#10156);
#8535=AXIS2_PLACEMENT_3D('',#12532,#10157,#10158);
#8536=AXIS2_PLACEMENT_3D('',#12533,#10159,#10160);
#8537=AXIS2_PLACEMENT_3D('',#12535,#10161,#10162);
#8538=AXIS2_PLACEMENT_3D('',#12537,#10164,#10165);
#8539=AXIS2_PLACEMENT_3D('',#12539,#10166,#10167);
#8540=AXIS2_PLACEMENT_3D('',#12545,#10171,#10172);
#8541=AXIS2_PLACEMENT_3D('',#12548,#10174,#10175);
#8542=AXIS2_PLACEMENT_3D('',#12549,#10176,#10177);
#8543=AXIS2_PLACEMENT_3D('',#12553,#10180,#10181);
#8544=AXIS2_PLACEMENT_3D('',#12557,#10184,#10185);
#8545=AXIS2_PLACEMENT_3D('',#12559,#10186,#10187);
#8546=AXIS2_PLACEMENT_3D('',#12562,#10189,#10190);
#8547=AXIS2_PLACEMENT_3D('',#12563,#10191,#10192);
#8548=AXIS2_PLACEMENT_3D('',#12565,#10193,#10194);
#8549=AXIS2_PLACEMENT_3D('',#12566,#10195,#10196);
#8550=AXIS2_PLACEMENT_3D('',#12568,#10197,#10198);
#8551=AXIS2_PLACEMENT_3D('',#12570,#10200,#10201);
#8552=AXIS2_PLACEMENT_3D('',#12572,#10202,#10203);
#8553=AXIS2_PLACEMENT_3D('',#12578,#10207,#10208);
#8554=AXIS2_PLACEMENT_3D('',#12581,#10210,#10211);
#8555=AXIS2_PLACEMENT_3D('',#12582,#10212,#10213);
#8556=AXIS2_PLACEMENT_3D('',#12588,#10217,#10218);
#8557=AXIS2_PLACEMENT_3D('',#12590,#10220,#10221);
#8558=AXIS2_PLACEMENT_3D('',#12592,#10222,#10223);
#8559=AXIS2_PLACEMENT_3D('',#12595,#10225,#10226);
#8560=AXIS2_PLACEMENT_3D('',#12596,#10227,#10228);
#8561=AXIS2_PLACEMENT_3D('',#12598,#10229,#10230);
#8562=AXIS2_PLACEMENT_3D('',#12599,#10231,#10232);
#8563=AXIS2_PLACEMENT_3D('',#12601,#10233,#10234);
#8564=AXIS2_PLACEMENT_3D('',#12603,#10236,#10237);
#8565=AXIS2_PLACEMENT_3D('',#12605,#10238,#10239);
#8566=AXIS2_PLACEMENT_3D('',#12614,#10244,#10245);
#8567=AXIS2_PLACEMENT_3D('',#12617,#10247,#10248);
#8568=AXIS2_PLACEMENT_3D('',#12618,#10249,#10250);
#8569=AXIS2_PLACEMENT_3D('',#12625,#10255,#10256);
#8570=AXIS2_PLACEMENT_3D('',#12629,#10259,#10260);
#8571=AXIS2_PLACEMENT_3D('',#12638,#10265,#10266);
#8572=AXIS2_PLACEMENT_3D('',#12644,#10270,#10271);
#8573=AXIS2_PLACEMENT_3D('',#12650,#10275,#10276);
#8574=AXIS2_PLACEMENT_3D('',#12653,#10279,#10280);
#8575=AXIS2_PLACEMENT_3D('',#12657,#10283,#10284);
#8576=AXIS2_PLACEMENT_3D('',#12658,#10285,#10286);
#8577=AXIS2_PLACEMENT_3D('',#12660,#10288,#10289);
#8578=AXIS2_PLACEMENT_3D('',#12664,#10292,#10293);
#8579=AXIS2_PLACEMENT_3D('',#12665,#10294,#10295);
#8580=AXIS2_PLACEMENT_3D('',#12666,#10296,#10297);
#8581=AXIS2_PLACEMENT_3D('',#12668,#10299,#10300);
#8582=AXIS2_PLACEMENT_3D('',#12669,#10301,#10302);
#8583=AXIS2_PLACEMENT_3D('',#12671,#10304,#10305);
#10100=DIRECTION('axis',(0.,0.,1.));
#10101=DIRECTION('refdir',(1.,0.,0.));
#10102=DIRECTION('center_axis',(0.,0.,1.));
#10103=DIRECTION('ref_axis',(1.,0.,0.));
#10104=DIRECTION('center_axis',(0.,0.,1.));
#10105=DIRECTION('ref_axis',(1.,0.,0.));
#10106=DIRECTION('',(0.,0.,1.));
#10107=DIRECTION('center_axis',(0.,0.,-1.));
#10108=DIRECTION('ref_axis',(1.,0.,0.));
#10109=DIRECTION('center_axis',(0.,0.,1.));
#10110=DIRECTION('ref_axis',(1.,0.,0.));
#10111=DIRECTION('center_axis',(0.,0.,1.));
#10112=DIRECTION('ref_axis',(1.,0.,0.));
#10113=DIRECTION('center_axis',(0.,0.,1.));
#10114=DIRECTION('ref_axis',(1.,0.,0.));
#10115=DIRECTION('center_axis',(0.,0.,1.));
#10116=DIRECTION('ref_axis',(1.,0.,0.));
#10117=DIRECTION('',(0.,0.,1.));
#10118=DIRECTION('center_axis',(0.,0.,1.));
#10119=DIRECTION('ref_axis',(1.,0.,0.));
#10120=DIRECTION('center_axis',(0.,0.,1.));
#10121=DIRECTION('ref_axis',(1.,0.,0.));
#10122=DIRECTION('',(0.,-1.,0.));
#10123=DIRECTION('',(-1.,0.,0.));
#10124=DIRECTION('',(0.,1.,0.));
#10125=DIRECTION('',(1.,0.,0.));
#10126=DIRECTION('center_axis',(0.,0.,1.));
#10127=DIRECTION('ref_axis',(1.,0.,0.));
#10128=DIRECTION('',(0.,0.,-1.));
#10129=DIRECTION('center_axis',(0.,0.,1.));
#10130=DIRECTION('ref_axis',(1.,0.,0.));
#10131=DIRECTION('center_axis',(1.,0.,0.));
#10132=DIRECTION('ref_axis',(0.,1.,0.));
#10133=DIRECTION('',(0.,0.,1.));
#10134=DIRECTION('',(0.,1.,0.));
#10135=DIRECTION('',(0.,0.,1.));
#10136=DIRECTION('',(0.,1.,0.));
#10137=DIRECTION('',(0.,0.,-1.));
#10138=DIRECTION('',(0.,1.,0.));
#10139=DIRECTION('',(0.,0.,1.));
#10140=DIRECTION('center_axis',(0.,1.,0.));
#10141=DIRECTION('ref_axis',(-1.,0.,0.));
#10142=DIRECTION('',(0.,0.,1.));
#10143=DIRECTION('',(-1.,0.,0.));
#10144=DIRECTION('',(0.,0.,-1.));
#10145=DIRECTION('',(-1.,0.,0.));
#10146=DIRECTION('',(0.,0.,1.));
#10147=DIRECTION('',(-1.,0.,0.));
#10148=DIRECTION('center_axis',(0.,0.,1.));
#10149=DIRECTION('ref_axis',(1.,0.,0.));
#10150=DIRECTION('center_axis',(0.,0.,1.));
#10151=DIRECTION('ref_axis',(1.,0.,0.));
#10152=DIRECTION('',(0.,0.,1.));
#10153=DIRECTION('center_axis',(0.,0.,-1.));
#10154=DIRECTION('ref_axis',(1.,0.,0.));
#10155=DIRECTION('center_axis',(0.,0.,1.));
#10156=DIRECTION('ref_axis',(1.,0.,0.));
#10157=DIRECTION('center_axis',(0.,0.,1.));
#10158=DIRECTION('ref_axis',(1.,0.,0.));
#10159=DIRECTION('center_axis',(0.,0.,1.));
#10160=DIRECTION('ref_axis',(1.,0.,0.));
#10161=DIRECTION('center_axis',(0.,0.,1.));
#10162=DIRECTION('ref_axis',(1.,0.,0.));
#10163=DIRECTION('',(0.,0.,1.));
#10164=DIRECTION('center_axis',(0.,0.,1.));
#10165=DIRECTION('ref_axis',(1.,0.,0.));
#10166=DIRECTION('center_axis',(0.,0.,1.));
#10167=DIRECTION('ref_axis',(1.,0.,0.));
#10168=DIRECTION('',(1.,0.,0.));
#10169=DIRECTION('',(0.,-1.,0.));
#10170=DIRECTION('',(-1.,0.,0.));
#10171=DIRECTION('center_axis',(0.,0.,1.));
#10172=DIRECTION('ref_axis',(1.,0.,0.));
#10173=DIRECTION('',(0.,0.,-1.));
#10174=DIRECTION('center_axis',(0.,0.,1.));
#10175=DIRECTION('ref_axis',(1.,0.,0.));
#10176=DIRECTION('center_axis',(0.,1.,0.));
#10177=DIRECTION('ref_axis',(0.,0.,1.));
#10178=DIRECTION('',(0.,0.,1.));
#10179=DIRECTION('',(-1.,0.,0.));
#10180=DIRECTION('center_axis',(-1.,0.,0.));
#10181=DIRECTION('ref_axis',(0.,0.,1.));
#10182=DIRECTION('',(0.,0.,-1.));
#10183=DIRECTION('',(0.,-1.,0.));
#10184=DIRECTION('center_axis',(0.,0.,1.));
#10185=DIRECTION('ref_axis',(1.,0.,0.));
#10186=DIRECTION('center_axis',(0.,0.,1.));
#10187=DIRECTION('ref_axis',(1.,0.,0.));
#10188=DIRECTION('',(0.,0.,1.));
#10189=DIRECTION('center_axis',(0.,0.,-1.));
#10190=DIRECTION('ref_axis',(1.,0.,0.));
#10191=DIRECTION('center_axis',(0.,0.,1.));
#10192=DIRECTION('ref_axis',(1.,0.,0.));
#10193=DIRECTION('center_axis',(0.,0.,1.));
#10194=DIRECTION('ref_axis',(1.,0.,0.));
#10195=DIRECTION('center_axis',(0.,0.,1.));
#10196=DIRECTION('ref_axis',(1.,0.,0.));
#10197=DIRECTION('center_axis',(0.,0.,1.));
#10198=DIRECTION('ref_axis',(1.,0.,0.));
#10199=DIRECTION('',(0.,0.,1.));
#10200=DIRECTION('center_axis',(0.,0.,1.));
#10201=DIRECTION('ref_axis',(1.,0.,0.));
#10202=DIRECTION('center_axis',(0.,0.,1.));
#10203=DIRECTION('ref_axis',(1.,0.,0.));
#10204=DIRECTION('',(0.,1.,0.));
#10205=DIRECTION('',(1.,0.,0.));
#10206=DIRECTION('',(0.,-1.,0.));
#10207=DIRECTION('center_axis',(0.,0.,1.));
#10208=DIRECTION('ref_axis',(1.,0.,0.));
#10209=DIRECTION('',(0.,0.,-1.));
#10210=DIRECTION('center_axis',(0.,0.,1.));
#10211=DIRECTION('ref_axis',(1.,0.,0.));
#10212=DIRECTION('center_axis',(0.,1.,0.));
#10213=DIRECTION('ref_axis',(1.,0.,0.));
#10214=DIRECTION('',(0.,0.,1.));
#10215=DIRECTION('',(1.,0.,0.));
#10216=DIRECTION('',(0.,0.,-1.));
#10217=DIRECTION('center_axis',(1.,0.,0.));
#10218=DIRECTION('ref_axis',(0.,0.,-1.));
#10219=DIRECTION('',(0.,1.,0.));
#10220=DIRECTION('center_axis',(0.,0.,1.));
#10221=DIRECTION('ref_axis',(1.,0.,0.));
#10222=DIRECTION('center_axis',(0.,0.,1.));
#10223=DIRECTION('ref_axis',(1.,0.,0.));
#10224=DIRECTION('',(0.,0.,1.));
#10225=DIRECTION('center_axis',(0.,0.,-1.));
#10226=DIRECTION('ref_axis',(1.,0.,0.));
#10227=DIRECTION('center_axis',(0.,0.,1.));
#10228=DIRECTION('ref_axis',(1.,0.,0.));
#10229=DIRECTION('center_axis',(0.,0.,1.));
#10230=DIRECTION('ref_axis',(1.,0.,0.));
#10231=DIRECTION('center_axis',(0.,0.,1.));
#10232=DIRECTION('ref_axis',(1.,0.,0.));
#10233=DIRECTION('center_axis',(0.,0.,1.));
#10234=DIRECTION('ref_axis',(1.,0.,0.));
#10235=DIRECTION('',(0.,0.,1.));
#10236=DIRECTION('center_axis',(0.,0.,1.));
#10237=DIRECTION('ref_axis',(1.,0.,0.));
#10238=DIRECTION('center_axis',(0.,0.,1.));
#10239=DIRECTION('ref_axis',(1.,0.,0.));
#10240=DIRECTION('',(-1.,0.,0.));
#10241=DIRECTION('',(0.,1.,0.));
#10242=DIRECTION('',(1.,0.,0.));
#10243=DIRECTION('',(0.,-1.,0.));
#10244=DIRECTION('center_axis',(0.,0.,1.));
#10245=DIRECTION('ref_axis',(1.,0.,0.));
#10246=DIRECTION('',(0.,0.,-1.));
#10247=DIRECTION('center_axis',(0.,0.,1.));
#10248=DIRECTION('ref_axis',(1.,0.,0.));
#10249=DIRECTION('center_axis',(0.,-1.,0.));
#10250=DIRECTION('ref_axis',(1.,0.,0.));
#10251=DIRECTION('',(1.,0.,0.));
#10252=DIRECTION('',(0.,0.,1.));
#10253=DIRECTION('',(0.,0.,1.));
#10254=DIRECTION('',(1.,0.,0.));
#10255=DIRECTION('center_axis',(1.,0.,0.));
#10256=DIRECTION('ref_axis',(0.,0.,-1.));
#10257=DIRECTION('',(0.,0.,-1.));
#10258=DIRECTION('',(0.,1.,0.));
#10259=DIRECTION('center_axis',(0.,-1.,0.));
#10260=DIRECTION('ref_axis',(1.,0.,0.));
#10261=DIRECTION('',(1.,0.,0.));
#10262=DIRECTION('',(0.,0.,1.));
#10263=DIRECTION('',(-1.,0.,0.));
#10264=DIRECTION('',(0.,0.,1.));
#10265=DIRECTION('center_axis',(1.,0.,0.));
#10266=DIRECTION('ref_axis',(0.,1.,0.));
#10267=DIRECTION('',(0.,1.,0.));
#10268=DIRECTION('',(0.,-1.,0.));
#10269=DIRECTION('',(0.,0.,1.));
#10270=DIRECTION('center_axis',(0.,1.,0.));
#10271=DIRECTION('ref_axis',(-1.,0.,0.));
#10272=DIRECTION('',(-1.,0.,0.));
#10273=DIRECTION('',(1.,0.,0.));
#10274=DIRECTION('',(0.,0.,1.));
#10275=DIRECTION('center_axis',(-1.,0.,0.));
#10276=DIRECTION('ref_axis',(0.,-1.,0.));
#10277=DIRECTION('',(0.,-1.,0.));
#10278=DIRECTION('',(0.,1.,0.));
#10279=DIRECTION('center_axis',(-1.,0.,0.));
#10280=DIRECTION('ref_axis',(0.,0.,1.));
#10281=DIRECTION('',(0.,0.,-1.));
#10282=DIRECTION('',(0.,-1.,0.));
#10283=DIRECTION('center_axis',(0.,0.,-1.));
#10284=DIRECTION('ref_axis',(-1.,0.,0.));
#10285=DIRECTION('center_axis',(0.,1.,0.));
#10286=DIRECTION('ref_axis',(1.,0.,0.));
#10287=DIRECTION('',(1.,0.,0.));
#10288=DIRECTION('center_axis',(0.,0.,1.));
#10289=DIRECTION('ref_axis',(1.,0.,0.));
#10290=DIRECTION('',(-1.,0.,0.));
#10291=DIRECTION('',(0.,-1.,0.));
#10292=DIRECTION('center_axis',(0.,0.,-1.));
#10293=DIRECTION('ref_axis',(-1.,0.,0.));
#10294=DIRECTION('center_axis',(0.,0.,-1.));
#10295=DIRECTION('ref_axis',(-1.,0.,0.));
#10296=DIRECTION('center_axis',(0.,1.,0.));
#10297=DIRECTION('ref_axis',(0.,0.,1.));
#10298=DIRECTION('',(0.,0.,1.));
#10299=DIRECTION('center_axis',(0.,0.,-1.));
#10300=DIRECTION('ref_axis',(-1.,0.,0.));
#10301=DIRECTION('center_axis',(-1.,0.,0.));
#10302=DIRECTION('ref_axis',(0.,-1.,0.));
#10303=DIRECTION('',(0.,-1.,0.));
#10304=DIRECTION('center_axis',(0.,0.,1.));
#10305=DIRECTION('ref_axis',(1.,0.,0.));
#12469=CARTESIAN_POINT('',(0.,0.,0.));
#12470=CARTESIAN_POINT('Origin',(4.4,3.4,1.5));
#12471=CARTESIAN_POINT('',(4.,3.4,1.5));
#12472=CARTESIAN_POINT('Origin',(4.4,3.4,1.5));
#12473=CARTESIAN_POINT('',(4.,3.4,11.5));
#12474=CARTESIAN_POINT('',(4.,3.4,1.5));
#12475=CARTESIAN_POINT('Origin',(4.4,3.4,11.5));
#12476=CARTESIAN_POINT('Origin',(4.4,3.4,1.5));
#12477=CARTESIAN_POINT('',(4.175,3.4,1.5));
#12478=CARTESIAN_POINT('Origin',(4.4,3.4,1.5));
#12479=CARTESIAN_POINT('Origin',(4.4,3.4,0.9));
#12480=CARTESIAN_POINT('',(4.175,3.4,1.));
#12481=CARTESIAN_POINT('Origin',(4.4,3.4,1.));
#12482=CARTESIAN_POINT('',(4.175,3.4,0.9));
#12483=CARTESIAN_POINT('Origin',(4.4,3.4,1.5));
#12484=CARTESIAN_POINT('',(3.5,3.4,1.5));
#12485=CARTESIAN_POINT('Origin',(4.4,3.4,1.5));
#12486=CARTESIAN_POINT('',(3.8,4.,1.5));
#12487=CARTESIAN_POINT('',(3.8,2.8,1.5));
#12488=CARTESIAN_POINT('',(3.8,3.1,1.5));
#12489=CARTESIAN_POINT('',(5.,4.,1.5));
#12490=CARTESIAN_POINT('',(4.7,4.,1.5));
#12491=CARTESIAN_POINT('',(5.,2.8,1.5));
#12492=CARTESIAN_POINT('',(5.,-0.3,1.5));
#12493=CARTESIAN_POINT('',(4.4,2.8,1.5));
#12494=CARTESIAN_POINT('Origin',(4.4,3.4,1.));
#12495=CARTESIAN_POINT('',(3.5,3.4,1.));
#12496=CARTESIAN_POINT('',(3.5,3.4,1.));
#12497=CARTESIAN_POINT('Origin',(4.4,3.4,1.));
#12498=CARTESIAN_POINT('Origin',(5.,-4.,11.));
#12499=CARTESIAN_POINT('',(5.,4.,11.5));
#12500=CARTESIAN_POINT('',(5.,4.,11.));
#12501=CARTESIAN_POINT('',(5.,-4.,11.5));
#12502=CARTESIAN_POINT('',(5.,-4.,11.5));
#12503=CARTESIAN_POINT('',(5.,-4.,1.5));
#12504=CARTESIAN_POINT('',(5.,-4.,11.));
#12505=CARTESIAN_POINT('',(5.,-2.8,1.5));
#12506=CARTESIAN_POINT('',(5.,-3.7,1.5));
#12507=CARTESIAN_POINT('',(5.,-2.8,11.));
#12508=CARTESIAN_POINT('',(5.,-2.8,1.));
#12509=CARTESIAN_POINT('',(5.,2.8,11.));
#12510=CARTESIAN_POINT('',(5.,-4.,11.));
#12511=CARTESIAN_POINT('',(5.,2.8,1.));
#12512=CARTESIAN_POINT('Origin',(5.,4.,11.));
#12513=CARTESIAN_POINT('',(3.8,4.,11.));
#12514=CARTESIAN_POINT('',(3.8,4.,11.2));
#12515=CARTESIAN_POINT('',(-3.8,4.,11.));
#12516=CARTESIAN_POINT('',(5.,4.,11.));
#12517=CARTESIAN_POINT('',(-3.8,4.,1.5));
#12518=CARTESIAN_POINT('',(-3.8,4.,1.));
#12519=CARTESIAN_POINT('',(-5.,4.,1.5));
#12520=CARTESIAN_POINT('',(0.3,4.,1.5));
#12521=CARTESIAN_POINT('',(-5.,4.,11.5));
#12522=CARTESIAN_POINT('',(-5.,4.,11.));
#12523=CARTESIAN_POINT('',(5.,4.,11.5));
#12524=CARTESIAN_POINT('Origin',(4.4,-3.4,1.5));
#12525=CARTESIAN_POINT('',(4.,-3.4,1.5));
#12526=CARTESIAN_POINT('Origin',(4.4,-3.4,1.5));
#12527=CARTESIAN_POINT('',(4.,-3.4,11.5));
#12528=CARTESIAN_POINT('',(4.,-3.4,1.5));
#12529=CARTESIAN_POINT('Origin',(4.4,-3.4,11.5));
#12530=CARTESIAN_POINT('Origin',(4.4,-3.4,1.5));
#12531=CARTESIAN_POINT('',(4.175,-3.4,1.5));
#12532=CARTESIAN_POINT('Origin',(4.4,-3.4,1.5));
#12533=CARTESIAN_POINT('Origin',(4.4,-3.4,0.9));
#12534=CARTESIAN_POINT('',(4.175,-3.4,1.));
#12535=CARTESIAN_POINT('Origin',(4.4,-3.4,1.));
#12536=CARTESIAN_POINT('',(4.175,-3.4,0.9));
#12537=CARTESIAN_POINT('Origin',(4.4,-3.4,1.5));
#12538=CARTESIAN_POINT('',(3.5,-3.4,1.5));
#12539=CARTESIAN_POINT('Origin',(4.4,-3.4,1.5));
#12540=CARTESIAN_POINT('',(3.8,-4.,1.5));
#12541=CARTESIAN_POINT('',(-0.3,-4.,1.5));
#12542=CARTESIAN_POINT('',(3.8,-2.8,1.5));
#12543=CARTESIAN_POINT('',(3.8,-3.7,1.5));
#12544=CARTESIAN_POINT('',(4.4,-2.8,1.5));
#12545=CARTESIAN_POINT('Origin',(4.4,-3.4,1.));
#12546=CARTESIAN_POINT('',(3.5,-3.4,1.));
#12547=CARTESIAN_POINT('',(3.5,-3.4,1.));
#12548=CARTESIAN_POINT('Origin',(4.4,-3.4,1.));
#12549=CARTESIAN_POINT('Origin',(4.4,-2.8,6.1));
#12550=CARTESIAN_POINT('',(3.8,-2.8,11.));
#12551=CARTESIAN_POINT('',(3.8,-2.8,11.2));
#12552=CARTESIAN_POINT('',(2.2,-2.8,11.));
#12553=CARTESIAN_POINT('Origin',(3.8,-4.,1.));
#12554=CARTESIAN_POINT('',(3.8,-4.,11.));
#12555=CARTESIAN_POINT('',(3.8,-4.,11.2));
#12556=CARTESIAN_POINT('',(3.8,-2.,11.));
#12557=CARTESIAN_POINT('Origin',(-4.4,3.4,1.5));
#12558=CARTESIAN_POINT('',(-4.8,3.4,1.5));
#12559=CARTESIAN_POINT('Origin',(-4.4,3.4,1.5));
#12560=CARTESIAN_POINT('',(-4.8,3.4,11.5));
#12561=CARTESIAN_POINT('',(-4.8,3.4,1.5));
#12562=CARTESIAN_POINT('Origin',(-4.4,3.4,11.5));
#12563=CARTESIAN_POINT('Origin',(-4.4,3.4,1.5));
#12564=CARTESIAN_POINT('',(-4.625,3.4,1.5));
#12565=CARTESIAN_POINT('Origin',(-4.4,3.4,1.5));
#12566=CARTESIAN_POINT('Origin',(-4.4,3.4,0.9));
#12567=CARTESIAN_POINT('',(-4.625,3.4,1.));
#12568=CARTESIAN_POINT('Origin',(-4.4,3.4,1.));
#12569=CARTESIAN_POINT('',(-4.625,3.4,0.9));
#12570=CARTESIAN_POINT('Origin',(-4.4,3.4,1.5));
#12571=CARTESIAN_POINT('',(-5.3,3.4,1.5));
#12572=CARTESIAN_POINT('Origin',(-4.4,3.4,1.5));
#12573=CARTESIAN_POINT('',(-3.8,2.8,1.5));
#12574=CARTESIAN_POINT('',(-3.8,3.1,1.5));
#12575=CARTESIAN_POINT('',(-5.,2.8,1.5));
#12576=CARTESIAN_POINT('',(-4.4,2.8,1.5));
#12577=CARTESIAN_POINT('',(-5.,3.7,1.5));
#12578=CARTESIAN_POINT('Origin',(-4.4,3.4,1.));
#12579=CARTESIAN_POINT('',(-5.3,3.4,1.));
#12580=CARTESIAN_POINT('',(-5.3,3.4,1.));
#12581=CARTESIAN_POINT('Origin',(-4.4,3.4,1.));
#12582=CARTESIAN_POINT('Origin',(-4.4,2.8,6.1));
#12583=CARTESIAN_POINT('',(-3.8,2.8,11.));
#12584=CARTESIAN_POINT('',(-3.8,2.8,1.));
#12585=CARTESIAN_POINT('',(-5.,2.8,11.));
#12586=CARTESIAN_POINT('',(-2.2,2.8,11.));
#12587=CARTESIAN_POINT('',(-5.,2.8,11.2));
#12588=CARTESIAN_POINT('Origin',(-3.8,2.8,11.2));
#12589=CARTESIAN_POINT('',(-3.8,1.4,11.));
#12590=CARTESIAN_POINT('Origin',(-4.4,-3.4,1.5));
#12591=CARTESIAN_POINT('',(-4.8,-3.4,1.5));
#12592=CARTESIAN_POINT('Origin',(-4.4,-3.4,1.5));
#12593=CARTESIAN_POINT('',(-4.8,-3.4,11.5));
#12594=CARTESIAN_POINT('',(-4.8,-3.4,1.5));
#12595=CARTESIAN_POINT('Origin',(-4.4,-3.4,11.5));
#12596=CARTESIAN_POINT('Origin',(-4.4,-3.4,1.5));
#12597=CARTESIAN_POINT('',(-4.625,-3.4,1.5));
#12598=CARTESIAN_POINT('Origin',(-4.4,-3.4,1.5));
#12599=CARTESIAN_POINT('Origin',(-4.4,-3.4,0.9));
#12600=CARTESIAN_POINT('',(-4.625,-3.4,1.));
#12601=CARTESIAN_POINT('Origin',(-4.4,-3.4,1.));
#12602=CARTESIAN_POINT('',(-4.625,-3.4,0.9));
#12603=CARTESIAN_POINT('Origin',(-4.4,-3.4,1.5));
#12604=CARTESIAN_POINT('',(-5.3,-3.4,1.5));
#12605=CARTESIAN_POINT('Origin',(-4.4,-3.4,1.5));
#12606=CARTESIAN_POINT('',(-3.8,-2.8,1.5));
#12607=CARTESIAN_POINT('',(-5.,-2.8,1.5));
#12608=CARTESIAN_POINT('',(-4.4,-2.8,1.5));
#12609=CARTESIAN_POINT('',(-3.8,-4.,1.5));
#12610=CARTESIAN_POINT('',(-3.8,-3.7,1.5));
#12611=CARTESIAN_POINT('',(-5.,-4.,1.5));
#12612=CARTESIAN_POINT('',(-4.7,-4.,1.5));
#12613=CARTESIAN_POINT('',(-5.,0.3,1.5));
#12614=CARTESIAN_POINT('Origin',(-4.4,-3.4,1.));
#12615=CARTESIAN_POINT('',(-5.3,-3.4,1.));
#12616=CARTESIAN_POINT('',(-5.3,-3.4,1.));
#12617=CARTESIAN_POINT('Origin',(-4.4,-3.4,1.));
#12618=CARTESIAN_POINT('Origin',(-5.,-4.,11.));
#12619=CARTESIAN_POINT('',(-5.,-4.,11.5));
#12620=CARTESIAN_POINT('',(-5.,-4.,11.5));
#12621=CARTESIAN_POINT('',(-5.,-4.,11.));
#12622=CARTESIAN_POINT('',(-3.8,-4.,11.));
#12623=CARTESIAN_POINT('',(-3.8,-4.,1.));
#12624=CARTESIAN_POINT('',(-5.,-4.,11.));
#12625=CARTESIAN_POINT('Origin',(-3.8,-4.,11.2));
#12626=CARTESIAN_POINT('',(-3.8,-2.8,11.));
#12627=CARTESIAN_POINT('',(-3.8,-2.8,1.));
#12628=CARTESIAN_POINT('',(-3.8,-2.,11.));
#12629=CARTESIAN_POINT('Origin',(-3.,-2.,10.9));
#12630=CARTESIAN_POINT('',(-3.,-2.,11.));
#12631=CARTESIAN_POINT('',(3.,-2.,11.));
#12632=CARTESIAN_POINT('',(-1.5,-2.,11.));
#12633=CARTESIAN_POINT('',(-3.,-2.,11.5));
#12634=CARTESIAN_POINT('',(-3.,-2.,10.9));
#12635=CARTESIAN_POINT('',(3.,-2.,11.5));
#12636=CARTESIAN_POINT('',(-1.5,-2.,11.5));
#12637=CARTESIAN_POINT('',(3.,-2.,10.9));
#12638=CARTESIAN_POINT('Origin',(3.,-2.,10.9));
#12639=CARTESIAN_POINT('',(3.,2.,11.));
#12640=CARTESIAN_POINT('',(3.,-1.,11.));
#12641=CARTESIAN_POINT('',(3.,2.,11.5));
#12642=CARTESIAN_POINT('',(3.,-1.,11.5));
#12643=CARTESIAN_POINT('',(3.,2.,10.9));
#12644=CARTESIAN_POINT('Origin',(3.,2.,10.9));
#12645=CARTESIAN_POINT('',(-3.,2.,11.));
#12646=CARTESIAN_POINT('',(1.5,2.,11.));
#12647=CARTESIAN_POINT('',(-3.,2.,11.5));
#12648=CARTESIAN_POINT('',(1.5,2.,11.5));
#12649=CARTESIAN_POINT('',(-3.,2.,10.9));
#12650=CARTESIAN_POINT('Origin',(-3.,2.,10.9));
#12651=CARTESIAN_POINT('',(-3.,1.,11.));
#12652=CARTESIAN_POINT('',(-3.,1.,11.5));
#12653=CARTESIAN_POINT('Origin',(3.8,2.8,1.));
#12654=CARTESIAN_POINT('',(3.8,2.8,11.));
#12655=CARTESIAN_POINT('',(3.8,2.8,11.2));
#12656=CARTESIAN_POINT('',(3.8,1.4,11.));
#12657=CARTESIAN_POINT('Origin',(5.,2.8,1.));
#12658=CARTESIAN_POINT('Origin',(4.4,2.8,6.1));
#12659=CARTESIAN_POINT('',(2.2,2.8,11.));
#12660=CARTESIAN_POINT('Origin',(0.,0.,11.));
#12661=CARTESIAN_POINT('',(-5.,-2.8,11.));
#12662=CARTESIAN_POINT('',(-2.2,-2.8,11.));
#12663=CARTESIAN_POINT('',(-5.,4.,11.));
#12664=CARTESIAN_POINT('Origin',(5.,-4.,1.));
#12665=CARTESIAN_POINT('Origin',(-3.8,2.8,1.));
#12666=CARTESIAN_POINT('Origin',(-4.4,-2.8,6.1));
#12667=CARTESIAN_POINT('',(-5.,-2.8,11.2));
#12668=CARTESIAN_POINT('Origin',(-3.8,-4.,1.));
#12669=CARTESIAN_POINT('Origin',(-5.,4.,11.));
#12670=CARTESIAN_POINT('',(-5.,4.,11.5));
#12671=CARTESIAN_POINT('Origin',(0.,0.,11.5));
#14747=UNCERTAINTY_MEASURE_WITH_UNIT(LENGTH_MEASURE(0.001),#14823,
'DISTANCE_ACCURACY_VALUE',
'Maximum model space distance between geometric entities at asserted c
onnectivities');
#14777=UNCERTAINTY_MEASURE_WITH_UNIT(LENGTH_MEASURE(0.001),#14823,
'DISTANCE_ACCURACY_VALUE',
'Maximum model space distance between geometric entities at asserted c
onnectivities');
#14792=(
GEOMETRIC_REPRESENTATION_CONTEXT(3)
GLOBAL_UNCERTAINTY_ASSIGNED_CONTEXT((#14747))
GLOBAL_UNIT_ASSIGNED_CONTEXT((#14823,#14825,#14826))
REPRESENTATION_CONTEXT('','3D')
);
#14822=(
GEOMETRIC_REPRESENTATION_CONTEXT(3)
GLOBAL_UNCERTAINTY_ASSIGNED_CONTEXT((#14777))
GLOBAL_UNIT_ASSIGNED_CONTEXT((#14823,#14825,#14826))
REPRESENTATION_CONTEXT('','3D')
);
#14823=(
LENGTH_UNIT()
NAMED_UNIT(*)
SI_UNIT(.CENTI.,.METRE.)
);
#14825=(
NAMED_UNIT(*)
PLANE_ANGLE_UNIT()
SI_UNIT($,.RADIAN.)
);
#14826=(
NAMED_UNIT(*)
SI_UNIT($,.STERADIAN.)
SOLID_ANGLE_UNIT()
);
#14841=SHAPE_DEFINITION_REPRESENTATION(#14885,#15012);
#14885=PRODUCT_DEFINITION_SHAPE('',$,#15057);
#15012=SHAPE_REPRESENTATION('',(#8517),#14792);
#15042=PRODUCT_DEFINITION_CONTEXT('part definition',#15176,'design');
#15057=PRODUCT_DEFINITION('Protective frame','Protective frame',#15101,
#15042);
#15101=PRODUCT_DEFINITION_FORMATION('',$,#15192);
#15176=APPLICATION_CONTEXT(
'Core Data for Automotive Mechanical Design Process');
#15177=PRODUCT_CONTEXT('part definition',#15176,'mechanical');
#15192=PRODUCT('Protective frame','Protective frame','Protective frame',
(#15177));
#15257=COLOUR_RGB('Dark Blue',0.08,0.2,0.34);
#15258=FILL_AREA_STYLE_COLOUR('',#15257);
#15259=FILL_AREA_STYLE('',(#15258));
#15260=SURFACE_STYLE_FILL_AREA(#15259);
#15261=SURFACE_SIDE_STYLE('',(#15260));
#15262=SURFACE_STYLE_USAGE(.BOTH.,#15261);
#15263=PRESENTATION_STYLE_ASSIGNMENT((#15262));
ENDSEC;
END-ISO-10303-21;
